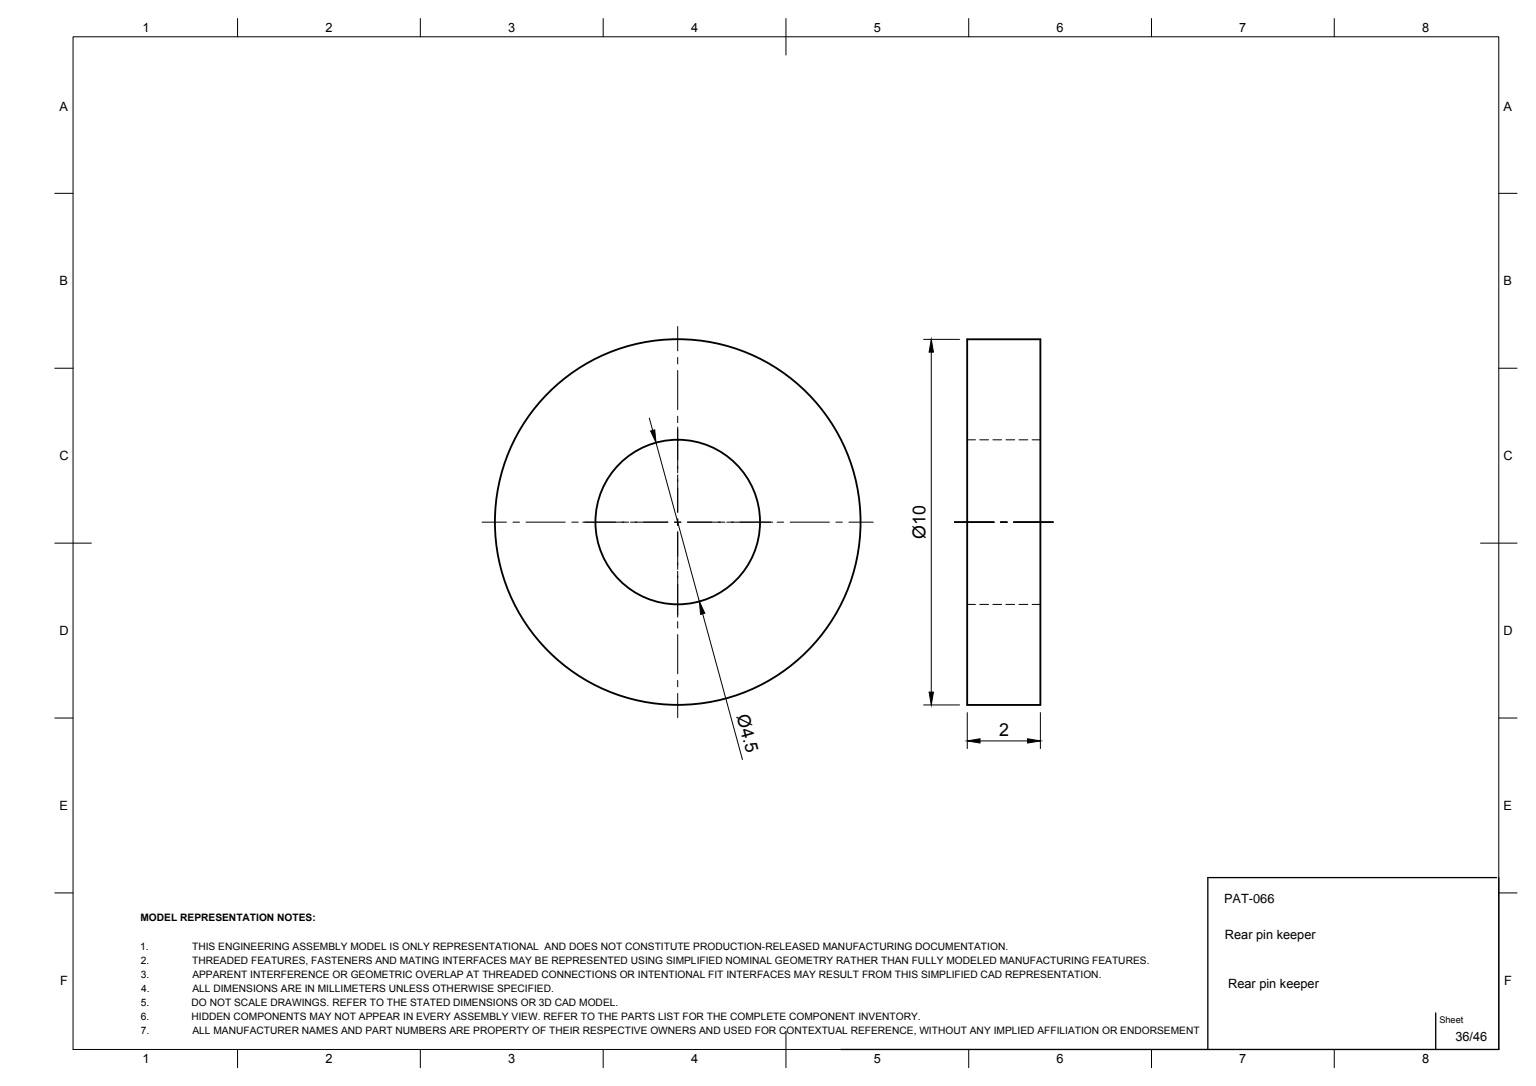
ISO-10303-21;
HEADER;
/* Generated by software containing ST-Developer
 * from STEP Tools, Inc. (www.steptools.com) 
 */

FILE_DESCRIPTION(
/* description */ ('Lever-operated bar clamp (toggle)'),
/* implementation_level */ '2;1');

FILE_NAME(
/* name */ 'Rear pin keeper.step',
/* time_stamp */ '2026-10-28T03:25:02-07:00',
/* author */ (''),
/* organization */ (''),
/* preprocessor_version */ 'ST-DEVELOPER v20.2',
/* originating_system */ 'Autodesk Translation Framework v15.17.0.0',
/* authorisation */ '');

FILE_SCHEMA (('AUTOMOTIVE_DESIGN { 1 0 10303 214 3 1 1 }'));
ENDSEC;

DATA;
#10=MECHANICAL_DESIGN_GEOMETRIC_PRESENTATION_REPRESENTATION('',(#445),#12413);
#361=SHAPE_REPRESENTATION_RELATIONSHIP('SRR','None',#12603,#399);
#399=ADVANCED_BREP_SHAPE_REPRESENTATION('',(#490),#12400);
#445=STYLED_ITEM('',(#12869),#490);
#490=MANIFOLD_SOLID_BREP('Body1',#6606);
#631=FACE_BOUND('',#1726,.T.);
#632=FACE_BOUND('',#1728,.T.);
#814=PLANE('',#7661);
#815=PLANE('',#7662);
#1186=FACE_OUTER_BOUND('',#1723,.T.);
#1187=FACE_OUTER_BOUND('',#1724,.T.);
#1188=FACE_OUTER_BOUND('',#1725,.T.);
#1189=FACE_OUTER_BOUND('',#1727,.T.);
#1723=EDGE_LOOP('',(#5611,#5612,#5613,#5614));
#1724=EDGE_LOOP('',(#5615,#5616,#5617,#5618));
#1725=EDGE_LOOP('',(#5619));
#1726=EDGE_LOOP('',(#5620));
#1727=EDGE_LOOP('',(#5621));
#1728=EDGE_LOOP('',(#5622));
#2146=LINE('',#11784,#2587);
#2147=LINE('',#11790,#2588);
#2587=VECTOR('',#9425,0.225);
#2588=VECTOR('',#9432,0.5);
#3011=CIRCLE('',#7656,0.225);
#3012=CIRCLE('',#7657,0.225);
#3013=CIRCLE('',#7659,0.5);
#3014=CIRCLE('',#7660,0.5);
#3478=VERTEX_POINT('',#11781);
#3479=VERTEX_POINT('',#11783);
#3480=VERTEX_POINT('',#11787);
#3481=VERTEX_POINT('',#11789);
#4210=EDGE_CURVE('',#3478,#3478,#3011,.T.);
#4211=EDGE_CURVE('',#3478,#3479,#2146,.T.);
#4212=EDGE_CURVE('',#3479,#3479,#3012,.T.);
#4213=EDGE_CURVE('',#3480,#3480,#3013,.T.);
#4214=EDGE_CURVE('',#3480,#3481,#2147,.T.);
#4215=EDGE_CURVE('',#3481,#3481,#3014,.T.);
#5611=ORIENTED_EDGE('',*,*,#4210,.F.);
#5612=ORIENTED_EDGE('',*,*,#4211,.T.);
#5613=ORIENTED_EDGE('',*,*,#4212,.T.);
#5614=ORIENTED_EDGE('',*,*,#4211,.F.);
#5615=ORIENTED_EDGE('',*,*,#4213,.F.);
#5616=ORIENTED_EDGE('',*,*,#4214,.T.);
#5617=ORIENTED_EDGE('',*,*,#4215,.T.);
#5618=ORIENTED_EDGE('',*,*,#4214,.F.);
#5619=ORIENTED_EDGE('',*,*,#4213,.T.);
#5620=ORIENTED_EDGE('',*,*,#4210,.T.);
#5621=ORIENTED_EDGE('',*,*,#4215,.F.);
#5622=ORIENTED_EDGE('',*,*,#4212,.F.);
#6139=CYLINDRICAL_SURFACE('',#7655,0.225);
#6140=CYLINDRICAL_SURFACE('',#7658,0.5);
#6461=ADVANCED_FACE('',(#1186),#6139,.F.);
#6462=ADVANCED_FACE('',(#1187),#6140,.T.);
#6463=ADVANCED_FACE('',(#1188,#631),#814,.T.);
#6464=ADVANCED_FACE('',(#1189,#632),#815,.F.);
#6606=CLOSED_SHELL('',(#6461,#6462,#6463,#6464));
#7654=AXIS2_PLACEMENT_3D('',#11779,#9419,#9420);
#7655=AXIS2_PLACEMENT_3D('',#11780,#9421,#9422);
#7656=AXIS2_PLACEMENT_3D('',#11782,#9423,#9424);
#7657=AXIS2_PLACEMENT_3D('',#11785,#9426,#9427);
#7658=AXIS2_PLACEMENT_3D('',#11786,#9428,#9429);
#7659=AXIS2_PLACEMENT_3D('',#11788,#9430,#9431);
#7660=AXIS2_PLACEMENT_3D('',#11791,#9433,#9434);
#7661=AXIS2_PLACEMENT_3D('',#11792,#9435,#9436);
#7662=AXIS2_PLACEMENT_3D('',#11793,#9437,#9438);
#9419=DIRECTION('axis',(0.,0.,1.));
#9420=DIRECTION('refdir',(1.,0.,0.));
#9421=DIRECTION('center_axis',(0.,1.,0.));
#9422=DIRECTION('ref_axis',(1.,0.,0.));
#9423=DIRECTION('center_axis',(0.,-1.,0.));
#9424=DIRECTION('ref_axis',(1.,0.,0.));
#9425=DIRECTION('',(0.,-1.,0.));
#9426=DIRECTION('center_axis',(0.,-1.,0.));
#9427=DIRECTION('ref_axis',(1.,0.,0.));
#9428=DIRECTION('center_axis',(0.,1.,0.));
#9429=DIRECTION('ref_axis',(1.,0.,0.));
#9430=DIRECTION('center_axis',(0.,1.,0.));
#9431=DIRECTION('ref_axis',(1.,0.,0.));
#9432=DIRECTION('',(0.,-1.,0.));
#9433=DIRECTION('center_axis',(0.,1.,0.));
#9434=DIRECTION('ref_axis',(1.,0.,0.));
#9435=DIRECTION('center_axis',(0.,1.,0.));
#9436=DIRECTION('ref_axis',(1.,0.,0.));
#9437=DIRECTION('center_axis',(0.,1.,0.));
#9438=DIRECTION('ref_axis',(1.,0.,0.));
#11779=CARTESIAN_POINT('',(0.,0.,0.));
#11780=CARTESIAN_POINT('Origin',(-2.82632109303527,-2.7,8.79263101785268));
#11781=CARTESIAN_POINT('',(-3.05132109303527,-2.5,8.79263101785268));
#11782=CARTESIAN_POINT('Origin',(-2.82632109303527,-2.5,8.79263101785268));
#11783=CARTESIAN_POINT('',(-3.05132109303527,-2.7,8.79263101785268));
#11784=CARTESIAN_POINT('',(-3.05132109303527,-2.7,8.79263101785268));
#11785=CARTESIAN_POINT('Origin',(-2.82632109303527,-2.7,8.79263101785268));
#11786=CARTESIAN_POINT('Origin',(-2.82632109303527,-2.7,8.79263101785268));
#11787=CARTESIAN_POINT('',(-3.32632109303527,-2.5,8.79263101785268));
#11788=CARTESIAN_POINT('Origin',(-2.82632109303527,-2.5,8.79263101785268));
#11789=CARTESIAN_POINT('',(-3.32632109303527,-2.7,8.79263101785268));
#11790=CARTESIAN_POINT('',(-3.32632109303527,-2.7,8.79263101785268));
#11791=CARTESIAN_POINT('Origin',(-2.82632109303527,-2.7,8.79263101785268));
#11792=CARTESIAN_POINT('Origin',(-2.82632109303527,-2.5,8.79263101785268));
#11793=CARTESIAN_POINT('Origin',(-2.82632109303527,-2.7,8.79263101785268));
#12354=UNCERTAINTY_MEASURE_WITH_UNIT(LENGTH_MEASURE(0.001),#12414,
'DISTANCE_ACCURACY_VALUE',
'Maximum model space distance between geometric entities at asserted c
onnectivities');
#12367=UNCERTAINTY_MEASURE_WITH_UNIT(LENGTH_MEASURE(0.001),#12414,
'DISTANCE_ACCURACY_VALUE',
'Maximum model space distance between geometric entities at asserted c
onnectivities');
#12400=(
GEOMETRIC_REPRESENTATION_CONTEXT(3)
GLOBAL_UNCERTAINTY_ASSIGNED_CONTEXT((#12354))
GLOBAL_UNIT_ASSIGNED_CONTEXT((#12414,#12416,#12417))
REPRESENTATION_CONTEXT('','3D')
);
#12413=(
GEOMETRIC_REPRESENTATION_CONTEXT(3)
GLOBAL_UNCERTAINTY_ASSIGNED_CONTEXT((#12367))
GLOBAL_UNIT_ASSIGNED_CONTEXT((#12414,#12416,#12417))
REPRESENTATION_CONTEXT('','3D')
);
#12414=(
LENGTH_UNIT()
NAMED_UNIT(*)
SI_UNIT(.CENTI.,.METRE.)
);
#12416=(
NAMED_UNIT(*)
PLANE_ANGLE_UNIT()
SI_UNIT($,.RADIAN.)
);
#12417=(
NAMED_UNIT(*)
SI_UNIT($,.STERADIAN.)
SOLID_ANGLE_UNIT()
);
#12450=SHAPE_DEFINITION_REPRESENTATION(#12502,#12603);
#12502=PRODUCT_DEFINITION_SHAPE('',$,#12649);
#12603=SHAPE_REPRESENTATION('',(#7654),#12400);
#12616=PRODUCT_DEFINITION_CONTEXT('part definition',#12753,'design');
#12649=PRODUCT_DEFINITION('Rear pin keeper','Rear pin keeper',#12694,#12616);
#12694=PRODUCT_DEFINITION_FORMATION('',$,#12787);
#12753=APPLICATION_CONTEXT(
'Core Data for Automotive Mechanical Design Process');
#12754=PRODUCT_CONTEXT('part definition',#12753,'mechanical');
#12787=PRODUCT('Rear pin keeper','Rear pin keeper','Rear pin keeper',(#12754));
#12863=COLOUR_RGB('Grey',0.48,0.52,0.57);
#12864=FILL_AREA_STYLE_COLOUR('',#12863);
#12865=FILL_AREA_STYLE('',(#12864));
#12866=SURFACE_STYLE_FILL_AREA(#12865);
#12867=SURFACE_SIDE_STYLE('',(#12866));
#12868=SURFACE_STYLE_USAGE(.BOTH.,#12867);
#12869=PRESENTATION_STYLE_ASSIGNMENT((#12868));
ENDSEC;
END-ISO-10303-21;
